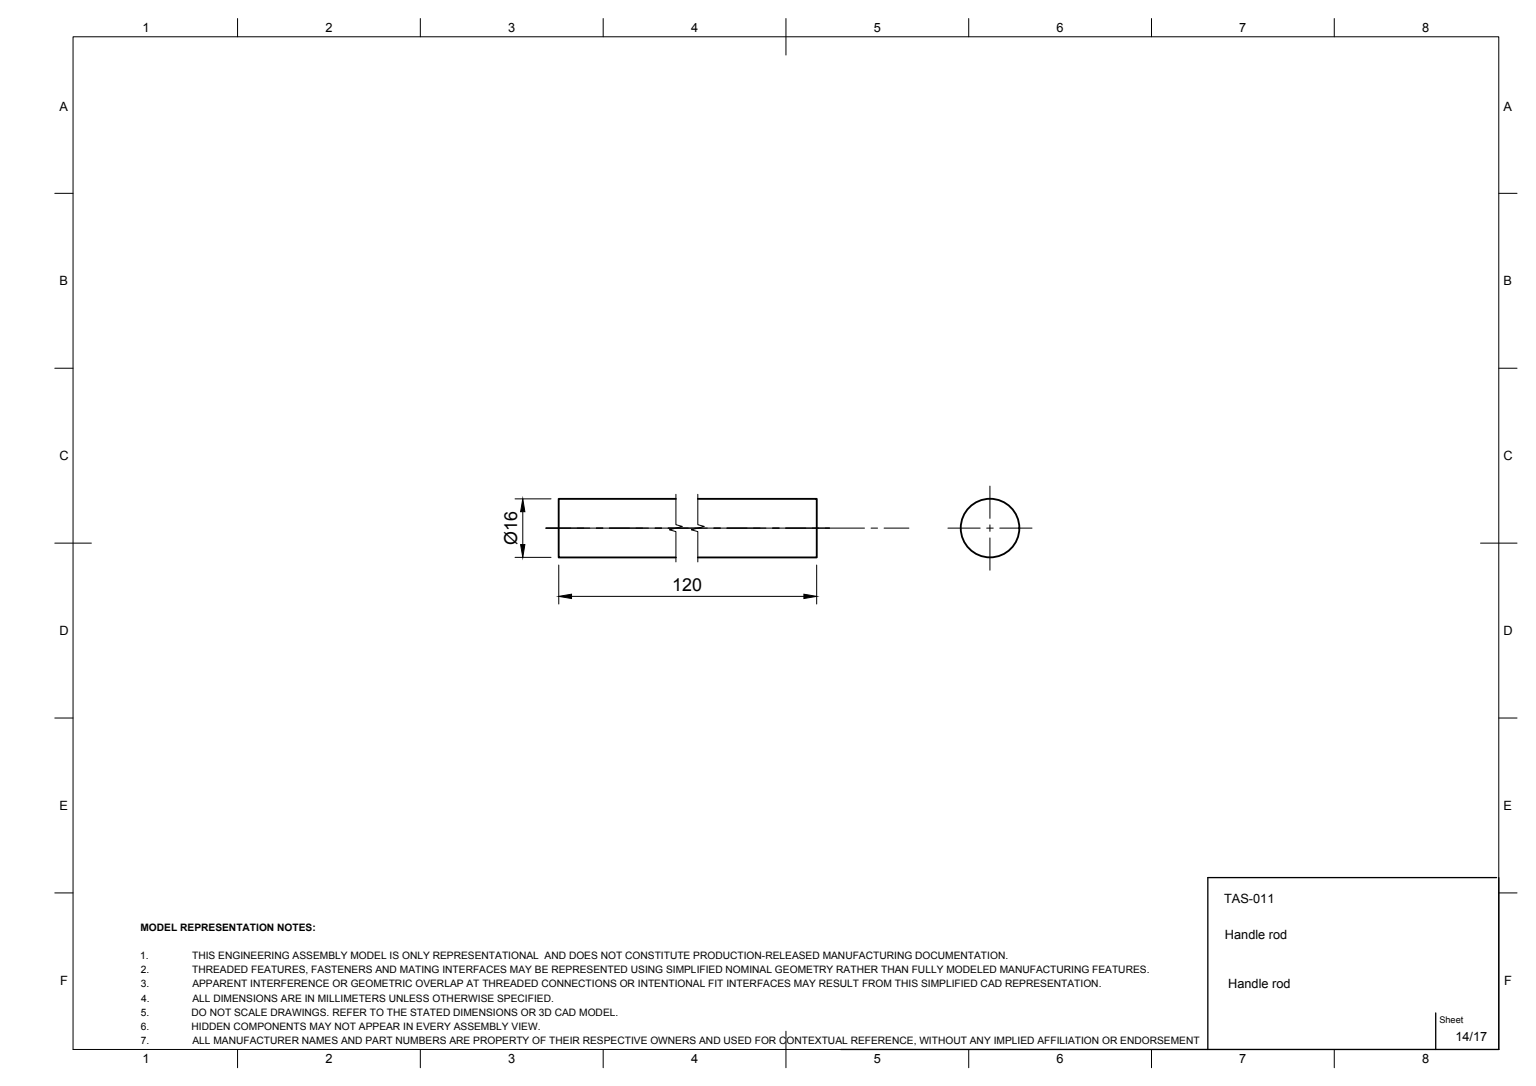
ISO-10303-21;
HEADER;
/* Generated by software containing ST-Developer
 * from STEP Tools, Inc. (www.steptools.com) 
 */

FILE_DESCRIPTION(
/* description */ (
'Independent manual bench leaf bending machine,200mm work width. Fabri
cated welded frame and folding leaf, repeated bushed and fully retaine
d hinge hardware, two handles with bonded grips, beveled clamping beam
 and modeledM12 clamp screws.2mm omitted-workpiece assembly reference 
gap, not a capacity claim. Native135deg hinge travel. Weld sizing, pro
duction fits, material condition, bending capacity, strength and life 
unassigned.'),
/* implementation_level */ '2;1');

FILE_NAME(
/* name */ 'Handle rod.step',
/* time_stamp */ '2026-11-14T09:11:34-08:00',
/* author */ (''),
/* organization */ (''),
/* preprocessor_version */ 'ST-DEVELOPER v20.2',
/* originating_system */ 'Autodesk Translation Framework v15.17.0.0',
/* authorisation */ '');

FILE_SCHEMA (('AUTOMOTIVE_DESIGN { 1 0 10303 214 3 1 1 }'));
ENDSEC;

DATA;
#10=MECHANICAL_DESIGN_GEOMETRIC_PRESENTATION_REPRESENTATION('',(#459),#37701);
#423=SHAPE_REPRESENTATION_RELATIONSHIP('SRR','None',#37792,#441);
#441=ADVANCED_BREP_SHAPE_REPRESENTATION('',(#477),#37696);
#459=STYLED_ITEM('',(#37884),#477);
#477=MANIFOLD_SOLID_BREP('Body1',#4157);
#586=PLANE('',#4623);
#587=PLANE('',#4624);
#787=FACE_OUTER_BOUND('',#1027,.T.);
#788=FACE_OUTER_BOUND('',#1028,.T.);
#789=FACE_OUTER_BOUND('',#1029,.T.);
#1027=EDGE_LOOP('',(#3733,#3734,#3735,#3736));
#1028=EDGE_LOOP('',(#3737));
#1029=EDGE_LOOP('',(#3738));
#1292=LINE('',#37536,#1541);
#1541=VECTOR('',#5461,8.);
#1615=CIRCLE('',#4621,8.);
#1616=CIRCLE('',#4622,8.);
#2027=VERTEX_POINT('',#37533);
#2028=VERTEX_POINT('',#37535);
#2600=EDGE_CURVE('',#2027,#2027,#1615,.T.);
#2601=EDGE_CURVE('',#2027,#2028,#1292,.T.);
#2602=EDGE_CURVE('',#2028,#2028,#1616,.T.);
#3733=ORIENTED_EDGE('',*,*,#2600,.F.);
#3734=ORIENTED_EDGE('',*,*,#2601,.T.);
#3735=ORIENTED_EDGE('',*,*,#2602,.T.);
#3736=ORIENTED_EDGE('',*,*,#2601,.F.);
#3737=ORIENTED_EDGE('',*,*,#2600,.T.);
#3738=ORIENTED_EDGE('',*,*,#2602,.F.);
#3921=CYLINDRICAL_SURFACE('',#4620,8.);
#4117=ADVANCED_FACE('',(#787),#3921,.T.);
#4118=ADVANCED_FACE('',(#788),#586,.T.);
#4119=ADVANCED_FACE('',(#789),#587,.F.);
#4157=CLOSED_SHELL('',(#4117,#4118,#4119));
#4619=AXIS2_PLACEMENT_3D('',#37531,#5455,#5456);
#4620=AXIS2_PLACEMENT_3D('',#37532,#5457,#5458);
#4621=AXIS2_PLACEMENT_3D('',#37534,#5459,#5460);
#4622=AXIS2_PLACEMENT_3D('',#37537,#5462,#5463);
#4623=AXIS2_PLACEMENT_3D('',#37538,#5464,#5465);
#4624=AXIS2_PLACEMENT_3D('',#37539,#5466,#5467);
#5455=DIRECTION('axis',(0.,0.,1.));
#5456=DIRECTION('refdir',(1.,0.,0.));
#5457=DIRECTION('center_axis',(0.,0.,1.));
#5458=DIRECTION('ref_axis',(1.,0.,0.));
#5459=DIRECTION('center_axis',(0.,0.,1.));
#5460=DIRECTION('ref_axis',(1.,0.,0.));
#5461=DIRECTION('',(0.,0.,-1.));
#5462=DIRECTION('center_axis',(0.,0.,1.));
#5463=DIRECTION('ref_axis',(1.,0.,0.));
#5464=DIRECTION('center_axis',(0.,0.,1.));
#5465=DIRECTION('ref_axis',(1.,0.,0.));
#5466=DIRECTION('center_axis',(0.,0.,1.));
#5467=DIRECTION('ref_axis',(1.,0.,0.));
#37531=CARTESIAN_POINT('',(0.,0.,0.));
#37532=CARTESIAN_POINT('Origin',(0.,0.,0.));
#37533=CARTESIAN_POINT('',(-8.,-9.79717439317883E-16,120.));
#37534=CARTESIAN_POINT('Origin',(0.,0.,120.));
#37535=CARTESIAN_POINT('',(-8.,-9.79717439317883E-16,0.));
#37536=CARTESIAN_POINT('',(-8.,-9.79717439317883E-16,0.));
#37537=CARTESIAN_POINT('Origin',(0.,0.,0.));
#37538=CARTESIAN_POINT('Origin',(0.,0.,120.));
#37539=CARTESIAN_POINT('Origin',(0.,0.,0.));
#37676=UNCERTAINTY_MEASURE_WITH_UNIT(LENGTH_MEASURE(0.01),#37702,
'DISTANCE_ACCURACY_VALUE',
'Maximum model space distance between geometric entities at asserted c
onnectivities');
#37681=UNCERTAINTY_MEASURE_WITH_UNIT(LENGTH_MEASURE(0.01),#37702,
'DISTANCE_ACCURACY_VALUE',
'Maximum model space distance between geometric entities at asserted c
onnectivities');
#37696=(
GEOMETRIC_REPRESENTATION_CONTEXT(3)
GLOBAL_UNCERTAINTY_ASSIGNED_CONTEXT((#37676))
GLOBAL_UNIT_ASSIGNED_CONTEXT((#37702,#37704,#37705))
REPRESENTATION_CONTEXT('','3D')
);
#37701=(
GEOMETRIC_REPRESENTATION_CONTEXT(3)
GLOBAL_UNCERTAINTY_ASSIGNED_CONTEXT((#37681))
GLOBAL_UNIT_ASSIGNED_CONTEXT((#37702,#37704,#37705))
REPRESENTATION_CONTEXT('','3D')
);
#37702=(
LENGTH_UNIT()
NAMED_UNIT(*)
SI_UNIT(.MILLI.,.METRE.)
);
#37704=(
NAMED_UNIT(*)
PLANE_ANGLE_UNIT()
SI_UNIT($,.RADIAN.)
);
#37705=(
NAMED_UNIT(*)
SI_UNIT($,.STERADIAN.)
SOLID_ANGLE_UNIT()
);
#37720=SHAPE_DEFINITION_REPRESENTATION(#37739,#37792);
#37739=PRODUCT_DEFINITION_SHAPE('',$,#37812);
#37792=SHAPE_REPRESENTATION('',(#4619),#37696);
#37797=PRODUCT_DEFINITION_CONTEXT('part definition',#37856,'design');
#37812=PRODUCT_DEFINITION('Handle rod','Handle rod',#37831,#37797);
#37831=PRODUCT_DEFINITION_FORMATION('',$,#37872);
#37856=APPLICATION_CONTEXT(
'Core Data for Automotive Mechanical Design Process');
#37857=PRODUCT_CONTEXT('part definition',#37856,'mechanical');
#37872=PRODUCT('Handle rod','Handle rod',$,(#37857));
#37884=PRESENTATION_STYLE_ASSIGNMENT((#37892));
#37892=SURFACE_STYLE_USAGE(.BOTH.,#37900);
#37900=SURFACE_SIDE_STYLE('',(#37908));
#37908=SURFACE_STYLE_FILL_AREA(#37916);
#37916=FILL_AREA_STYLE('Opaque(147,157,170)',(#37924));
#37924=FILL_AREA_STYLE_COLOUR('Opaque(147,157,170)',#37932);
#37932=COLOUR_RGB('Opaque(147,157,170)',0.576470588235294,0.615686274509804,
0.666666666666667);
ENDSEC;
END-ISO-10303-21;
